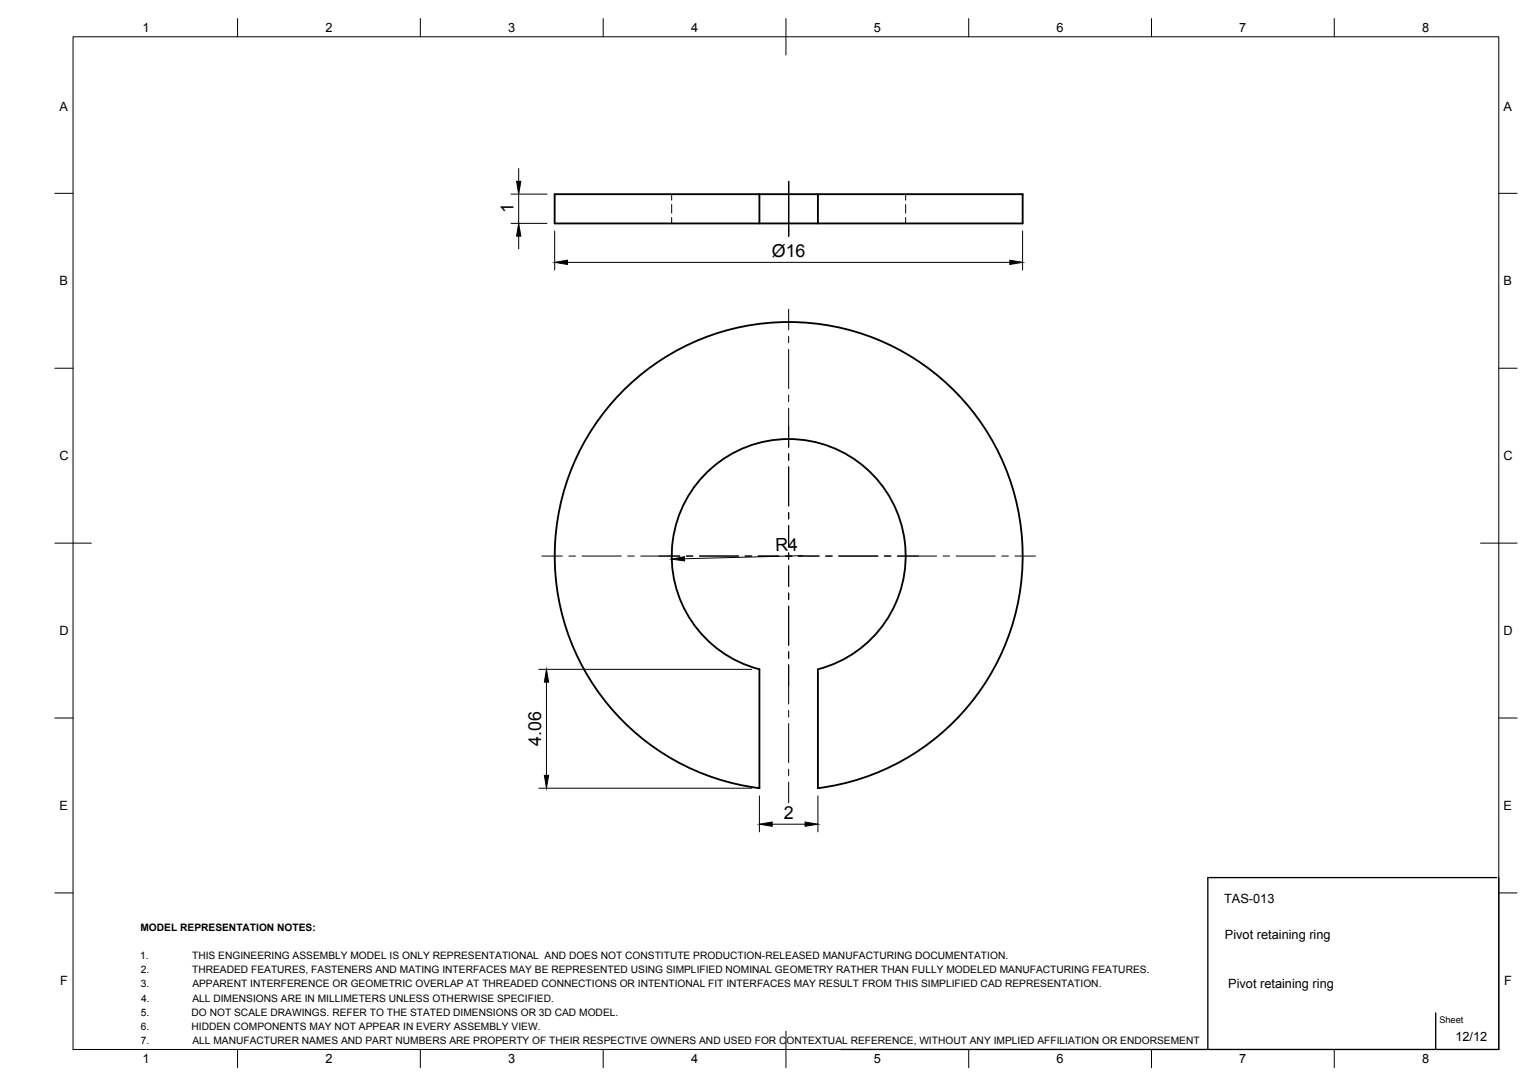
ISO-10303-21;
HEADER;
/* Generated by software containing ST-Developer
 * from STEP Tools, Inc. (www.steptools.com) 
 */

FILE_DESCRIPTION(
/* description */ (
'Independent guided parallel-jaw bracket clamp. Two12mm guide rods, re
placeable bronze sleeves, captured swiveling spindle, replaceable jaw 
pads and modeled M16x2 screw. Native slider/revolute joints linked2mm 
per revolution. Nominal opening0..122 with initial28mm. Base and two i
dentical supports welded. Standard fits, weld details and clamp load r
equire engineering selection.'),
/* implementation_level */ '2;1');

FILE_NAME(
/* name */ 'Pivot retaining ring.step',
/* time_stamp */ '2026-11-14T09:15:44-08:00',
/* author */ (''),
/* organization */ (''),
/* preprocessor_version */ 'ST-DEVELOPER v20.2',
/* originating_system */ 'Autodesk Translation Framework v15.17.0.0',
/* authorisation */ '');

FILE_SCHEMA (('AUTOMOTIVE_DESIGN { 1 0 10303 214 3 1 1 }'));
ENDSEC;

DATA;
#10=MECHANICAL_DESIGN_GEOMETRIC_PRESENTATION_REPRESENTATION('',(#919),#105806);
#895=SHAPE_REPRESENTATION_RELATIONSHIP('SRR','None',#105863,#907);
#907=ADVANCED_BREP_SHAPE_REPRESENTATION('',(#931),#105798);
#919=STYLED_ITEM('',(#105932),#931);
#931=MANIFOLD_SOLID_BREP('Body1',#7206);
#1026=PLANE('',#7528);
#1027=PLANE('',#7529);
#1028=PLANE('',#7530);
#1029=PLANE('',#7537);
#1195=FACE_OUTER_BOUND('',#1501,.T.);
#1196=FACE_OUTER_BOUND('',#1502,.T.);
#1197=FACE_OUTER_BOUND('',#1503,.T.);
#1198=FACE_OUTER_BOUND('',#1504,.T.);
#1199=FACE_OUTER_BOUND('',#1505,.T.);
#1200=FACE_OUTER_BOUND('',#1506,.T.);
#1501=EDGE_LOOP('',(#5695,#5696,#5697,#5698));
#1502=EDGE_LOOP('',(#5699,#5700,#5701,#5702));
#1503=EDGE_LOOP('',(#5703,#5704,#5705,#5706));
#1504=EDGE_LOOP('',(#5707,#5708,#5709,#5710));
#1505=EDGE_LOOP('',(#5711,#5712,#5713,#5714));
#1506=EDGE_LOOP('',(#5715,#5716,#5717,#5718));
#1807=LINE('',#71874,#2087);
#1808=LINE('',#71876,#2088);
#1809=LINE('',#71878,#2089);
#1810=LINE('',#71879,#2090);
#1811=LINE('',#71883,#2091);
#1812=LINE('',#71885,#2092);
#1813=LINE('',#71887,#2093);
#1814=LINE('',#71888,#2094);
#2087=VECTOR('',#8246,10.);
#2088=VECTOR('',#8247,10.);
#2089=VECTOR('',#8248,10.);
#2090=VECTOR('',#8249,10.);
#2091=VECTOR('',#8252,10.);
#2092=VECTOR('',#8253,10.);
#2093=VECTOR('',#8254,10.);
#2094=VECTOR('',#8255,10.);
#2273=CIRCLE('',#7531,8.);
#2274=CIRCLE('',#7532,4.);
#2275=CIRCLE('',#7534,4.);
#2276=CIRCLE('',#7536,8.);
#2851=VERTEX_POINT('',#71872);
#2852=VERTEX_POINT('',#71873);
#2853=VERTEX_POINT('',#71875);
#2854=VERTEX_POINT('',#71877);
#2855=VERTEX_POINT('',#71881);
#2856=VERTEX_POINT('',#71882);
#2857=VERTEX_POINT('',#71884);
#2858=VERTEX_POINT('',#71886);
#3892=EDGE_CURVE('',#2851,#2852,#1807,.T.);
#3893=EDGE_CURVE('',#2853,#2851,#1808,.T.);
#3894=EDGE_CURVE('',#2854,#2853,#1809,.T.);
#3895=EDGE_CURVE('',#2852,#2854,#1810,.T.);
#3896=EDGE_CURVE('',#2855,#2856,#1811,.T.);
#3897=EDGE_CURVE('',#2857,#2855,#1812,.T.);
#3898=EDGE_CURVE('',#2858,#2857,#1813,.T.);
#3899=EDGE_CURVE('',#2856,#2858,#1814,.T.);
#3900=EDGE_CURVE('',#2853,#2858,#2273,.T.);
#3901=EDGE_CURVE('',#2856,#2851,#2274,.T.);
#3902=EDGE_CURVE('',#2855,#2852,#2275,.T.);
#3903=EDGE_CURVE('',#2854,#2857,#2276,.T.);
#5695=ORIENTED_EDGE('',*,*,#3892,.F.);
#5696=ORIENTED_EDGE('',*,*,#3893,.F.);
#5697=ORIENTED_EDGE('',*,*,#3894,.F.);
#5698=ORIENTED_EDGE('',*,*,#3895,.F.);
#5699=ORIENTED_EDGE('',*,*,#3896,.F.);
#5700=ORIENTED_EDGE('',*,*,#3897,.F.);
#5701=ORIENTED_EDGE('',*,*,#3898,.F.);
#5702=ORIENTED_EDGE('',*,*,#3899,.F.);
#5703=ORIENTED_EDGE('',*,*,#3899,.T.);
#5704=ORIENTED_EDGE('',*,*,#3900,.F.);
#5705=ORIENTED_EDGE('',*,*,#3893,.T.);
#5706=ORIENTED_EDGE('',*,*,#3901,.F.);
#5707=ORIENTED_EDGE('',*,*,#3896,.T.);
#5708=ORIENTED_EDGE('',*,*,#3901,.T.);
#5709=ORIENTED_EDGE('',*,*,#3892,.T.);
#5710=ORIENTED_EDGE('',*,*,#3902,.F.);
#5711=ORIENTED_EDGE('',*,*,#3898,.T.);
#5712=ORIENTED_EDGE('',*,*,#3903,.F.);
#5713=ORIENTED_EDGE('',*,*,#3894,.T.);
#5714=ORIENTED_EDGE('',*,*,#3900,.T.);
#5715=ORIENTED_EDGE('',*,*,#3897,.T.);
#5716=ORIENTED_EDGE('',*,*,#3902,.T.);
#5717=ORIENTED_EDGE('',*,*,#3895,.T.);
#5718=ORIENTED_EDGE('',*,*,#3903,.T.);
#6836=CYLINDRICAL_SURFACE('',#7533,4.);
#6837=CYLINDRICAL_SURFACE('',#7535,8.);
#7060=ADVANCED_FACE('',(#1195),#1026,.F.);
#7061=ADVANCED_FACE('',(#1196),#1027,.F.);
#7062=ADVANCED_FACE('',(#1197),#1028,.F.);
#7063=ADVANCED_FACE('',(#1198),#6836,.F.);
#7064=ADVANCED_FACE('',(#1199),#6837,.T.);
#7065=ADVANCED_FACE('',(#1200),#1029,.T.);
#7206=CLOSED_SHELL('',(#7060,#7061,#7062,#7063,#7064,#7065));
#7527=AXIS2_PLACEMENT_3D('',#71870,#8242,#8243);
#7528=AXIS2_PLACEMENT_3D('',#71871,#8244,#8245);
#7529=AXIS2_PLACEMENT_3D('',#71880,#8250,#8251);
#7530=AXIS2_PLACEMENT_3D('',#71889,#8256,#8257);
#7531=AXIS2_PLACEMENT_3D('',#71890,#8258,#8259);
#7532=AXIS2_PLACEMENT_3D('',#71891,#8260,#8261);
#7533=AXIS2_PLACEMENT_3D('',#71892,#8262,#8263);
#7534=AXIS2_PLACEMENT_3D('',#71893,#8264,#8265);
#7535=AXIS2_PLACEMENT_3D('',#71894,#8266,#8267);
#7536=AXIS2_PLACEMENT_3D('',#71895,#8268,#8269);
#7537=AXIS2_PLACEMENT_3D('',#71896,#8270,#8271);
#8242=DIRECTION('axis',(0.,0.,1.));
#8243=DIRECTION('refdir',(1.,0.,0.));
#8244=DIRECTION('center_axis',(-1.,0.,0.));
#8245=DIRECTION('ref_axis',(0.,1.,0.));
#8246=DIRECTION('',(0.,0.,1.));
#8247=DIRECTION('',(0.,-1.,0.));
#8248=DIRECTION('',(0.,0.,-1.));
#8249=DIRECTION('',(0.,1.,0.));
#8250=DIRECTION('center_axis',(1.,0.,0.));
#8251=DIRECTION('ref_axis',(0.,-1.,0.));
#8252=DIRECTION('',(0.,0.,-1.));
#8253=DIRECTION('',(0.,-1.,0.));
#8254=DIRECTION('',(0.,0.,1.));
#8255=DIRECTION('',(0.,1.,0.));
#8256=DIRECTION('center_axis',(0.,0.,1.));
#8257=DIRECTION('ref_axis',(1.,0.,0.));
#8258=DIRECTION('center_axis',(0.,0.,1.));
#8259=DIRECTION('ref_axis',(1.,0.,0.));
#8260=DIRECTION('center_axis',(0.,0.,-1.));
#8261=DIRECTION('ref_axis',(1.,0.,0.));
#8262=DIRECTION('center_axis',(0.,0.,1.));
#8263=DIRECTION('ref_axis',(6.12323399573677E-17,-1.,0.));
#8264=DIRECTION('center_axis',(0.,0.,-1.));
#8265=DIRECTION('ref_axis',(1.,0.,0.));
#8266=DIRECTION('center_axis',(0.,0.,1.));
#8267=DIRECTION('ref_axis',(6.12323399573677E-17,-1.,0.));
#8268=DIRECTION('center_axis',(0.,0.,1.));
#8269=DIRECTION('ref_axis',(1.,0.,0.));
#8270=DIRECTION('center_axis',(0.,0.,1.));
#8271=DIRECTION('ref_axis',(1.,0.,0.));
#71870=CARTESIAN_POINT('',(0.,0.,0.));
#71871=CARTESIAN_POINT('Origin',(-1.,0.,1.));
#71872=CARTESIAN_POINT('',(-1.,3.87298334620742,0.));
#71873=CARTESIAN_POINT('',(-1.,3.87298334620742,1.));
#71874=CARTESIAN_POINT('',(-1.,3.87298334620742,0.));
#71875=CARTESIAN_POINT('',(-1.,7.93725393319377,0.));
#71876=CARTESIAN_POINT('',(-1.,0.,0.));
#71877=CARTESIAN_POINT('',(-1.,7.93725393319377,1.));
#71878=CARTESIAN_POINT('',(-1.,7.93725393319377,0.));
#71879=CARTESIAN_POINT('',(-1.,0.,1.));
#71880=CARTESIAN_POINT('Origin',(1.,16.,1.));
#71881=CARTESIAN_POINT('',(1.,3.87298334620742,1.));
#71882=CARTESIAN_POINT('',(1.,3.87298334620742,0.));
#71883=CARTESIAN_POINT('',(1.,3.87298334620742,0.));
#71884=CARTESIAN_POINT('',(1.,7.93725393319377,1.));
#71885=CARTESIAN_POINT('',(1.,8.,1.));
#71886=CARTESIAN_POINT('',(1.,7.93725393319377,0.));
#71887=CARTESIAN_POINT('',(1.,7.93725393319377,0.));
#71888=CARTESIAN_POINT('',(1.,8.,0.));
#71889=CARTESIAN_POINT('Origin',(0.,0.,0.));
#71890=CARTESIAN_POINT('Origin',(0.,0.,0.));
#71891=CARTESIAN_POINT('Origin',(0.,0.,0.));
#71892=CARTESIAN_POINT('Origin',(0.,0.,0.));
#71893=CARTESIAN_POINT('Origin',(0.,0.,1.));
#71894=CARTESIAN_POINT('Origin',(0.,0.,0.));
#71895=CARTESIAN_POINT('Origin',(0.,0.,1.));
#71896=CARTESIAN_POINT('Origin',(0.,0.,1.));
#105784=UNCERTAINTY_MEASURE_WITH_UNIT(LENGTH_MEASURE(0.01),#105807,
'DISTANCE_ACCURACY_VALUE',
'Maximum model space distance between geometric entities at asserted c
onnectivities');
#105792=UNCERTAINTY_MEASURE_WITH_UNIT(LENGTH_MEASURE(0.01),#105807,
'DISTANCE_ACCURACY_VALUE',
'Maximum model space distance between geometric entities at asserted c
onnectivities');
#105798=(
GEOMETRIC_REPRESENTATION_CONTEXT(3)
GLOBAL_UNCERTAINTY_ASSIGNED_CONTEXT((#105784))
GLOBAL_UNIT_ASSIGNED_CONTEXT((#105807,#105809,#105810))
REPRESENTATION_CONTEXT('','3D')
);
#105806=(
GEOMETRIC_REPRESENTATION_CONTEXT(3)
GLOBAL_UNCERTAINTY_ASSIGNED_CONTEXT((#105792))
GLOBAL_UNIT_ASSIGNED_CONTEXT((#105807,#105809,#105810))
REPRESENTATION_CONTEXT('','3D')
);
#105807=(
LENGTH_UNIT()
NAMED_UNIT(*)
SI_UNIT(.MILLI.,.METRE.)
);
#105809=(
NAMED_UNIT(*)
PLANE_ANGLE_UNIT()
SI_UNIT($,.RADIAN.)
);
#105810=(
NAMED_UNIT(*)
SI_UNIT($,.STERADIAN.)
SOLID_ANGLE_UNIT()
);
#105816=SHAPE_DEFINITION_REPRESENTATION(#105829,#105863);
#105829=PRODUCT_DEFINITION_SHAPE('',$,#105877);
#105863=SHAPE_REPRESENTATION('',(#7527),#105798);
#105871=PRODUCT_DEFINITION_CONTEXT('part definition',#105912,'design');
#105877=PRODUCT_DEFINITION('Pivot retaining ring',
'Pivot retaining ring',#105890,#105871);
#105890=PRODUCT_DEFINITION_FORMATION('',$,#105919);
#105912=APPLICATION_CONTEXT(
'Core Data for Automotive Mechanical Design Process');
#105913=PRODUCT_CONTEXT('part definition',#105912,'mechanical');
#105919=PRODUCT('Pivot retaining ring','Pivot retaining ring',$,(#105913));
#105932=PRESENTATION_STYLE_ASSIGNMENT((#105938));
#105938=SURFACE_STYLE_USAGE(.BOTH.,#105944);
#105944=SURFACE_SIDE_STYLE('',(#105950));
#105950=SURFACE_STYLE_FILL_AREA(#105956);
#105956=FILL_AREA_STYLE('Opaque(64,72,82)',(#105962));
#105962=FILL_AREA_STYLE_COLOUR('Opaque(64,72,82)',#105968);
#105968=COLOUR_RGB('Opaque(64,72,82)',0.250980392156863,0.282352941176471,
0.32156862745098);
ENDSEC;
END-ISO-10303-21;
